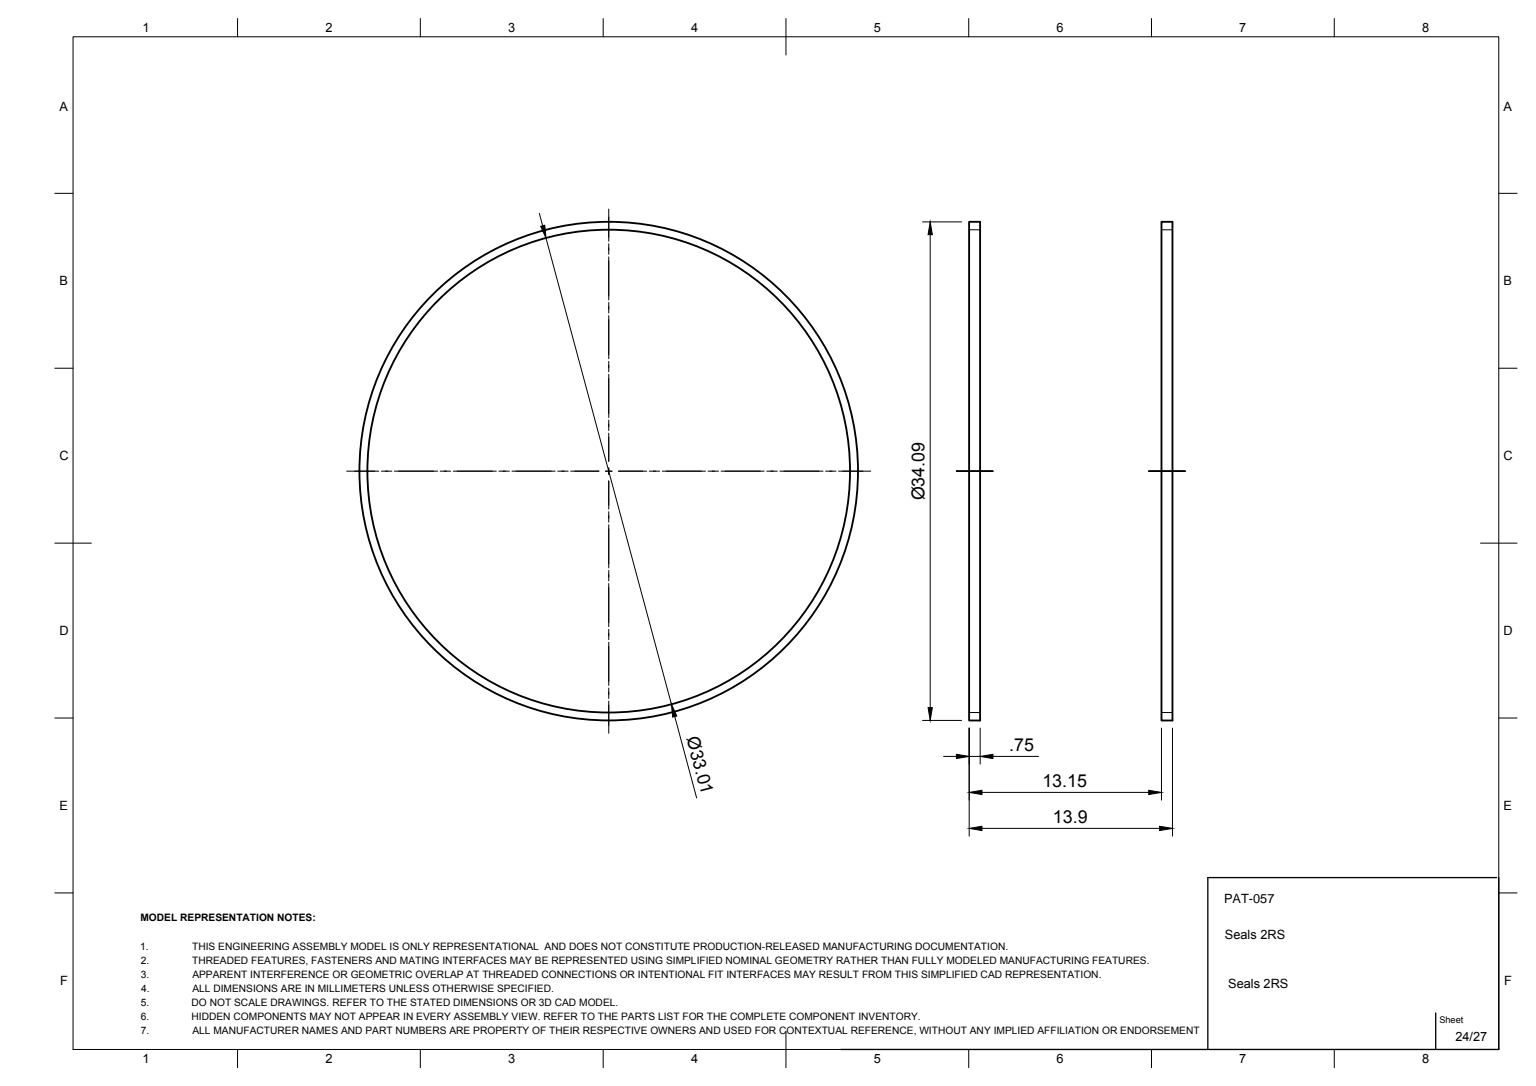
ISO-10303-21;
HEADER;
/* Generated by software containing ST-Developer
 * from STEP Tools, Inc. (www.steptools.com) 
 */

FILE_DESCRIPTION(
/* description */ ('Bearing-mounted hook block'),
/* implementation_level */ '2;1');

FILE_NAME(
/* name */ 'Seals 2RS.step',
/* time_stamp */ '2026-10-28T22:30:11-07:00',
/* author */ (''),
/* organization */ (''),
/* preprocessor_version */ 'ST-DEVELOPER v20.2',
/* originating_system */ 'Autodesk Translation Framework v15.17.0.0',
/* authorisation */ '');

FILE_SCHEMA (('AUTOMOTIVE_DESIGN { 1 0 10303 214 3 1 1 }'));
ENDSEC;

DATA;
#10=MECHANICAL_DESIGN_GEOMETRIC_PRESENTATION_REPRESENTATION('',(#348,#349),#7609);
#293=SHAPE_REPRESENTATION_RELATIONSHIP('SRR','None',#7742,#317);
#317=ADVANCED_BREP_SHAPE_REPRESENTATION('',(#378,#379),#7602);
#348=STYLED_ITEM('',(#7931),#378);
#349=STYLED_ITEM('',(#7931),#379);
#378=MANIFOLD_SOLID_BREP('Body1',#3946);
#379=MANIFOLD_SOLID_BREP('Body2',#3947);
#537=LINE('',#7259,#767);
#538=LINE('',#7264,#768);
#539=LINE('',#7273,#769);
#540=LINE('',#7278,#770);
#767=VECTOR('',#5714,1.70469);
#768=VECTOR('',#5721,1.65031);
#769=VECTOR('',#5732,1.70469);
#770=VECTOR('',#5739,1.65031);
#900=CYLINDRICAL_SURFACE('',#4619,1.70469);
#901=CYLINDRICAL_SURFACE('',#4623,1.65031);
#902=CYLINDRICAL_SURFACE('',#4627,1.70469);
#903=CYLINDRICAL_SURFACE('',#4631,1.65031);
#979=FACE_BOUND('',#1469,.T.);
#980=FACE_BOUND('',#1472,.T.);
#981=FACE_BOUND('',#1475,.T.);
#982=FACE_BOUND('',#1478,.T.);
#1174=FACE_OUTER_BOUND('',#1468,.T.);
#1175=FACE_OUTER_BOUND('',#1470,.T.);
#1176=FACE_OUTER_BOUND('',#1471,.T.);
#1177=FACE_OUTER_BOUND('',#1473,.T.);
#1178=FACE_OUTER_BOUND('',#1474,.T.);
#1179=FACE_OUTER_BOUND('',#1476,.T.);
#1180=FACE_OUTER_BOUND('',#1477,.T.);
#1181=FACE_OUTER_BOUND('',#1479,.T.);
#1468=EDGE_LOOP('',(#3312));
#1469=EDGE_LOOP('',(#3313));
#1470=EDGE_LOOP('',(#3314,#3315,#3316,#3317));
#1471=EDGE_LOOP('',(#3318));
#1472=EDGE_LOOP('',(#3319));
#1473=EDGE_LOOP('',(#3320,#3321,#3322,#3323));
#1474=EDGE_LOOP('',(#3324));
#1475=EDGE_LOOP('',(#3325));
#1476=EDGE_LOOP('',(#3326,#3327,#3328,#3329));
#1477=EDGE_LOOP('',(#3330));
#1478=EDGE_LOOP('',(#3331));
#1479=EDGE_LOOP('',(#3332,#3333,#3334,#3335));
#1731=CIRCLE('',#4617,1.70469);
#1732=CIRCLE('',#4618,1.65031);
#1733=CIRCLE('',#4620,1.70469);
#1734=CIRCLE('',#4622,1.65031);
#1735=CIRCLE('',#4625,1.70469);
#1736=CIRCLE('',#4626,1.65031);
#1737=CIRCLE('',#4628,1.70469);
#1738=CIRCLE('',#4630,1.65031);
#2024=VERTEX_POINT('',#7252);
#2025=VERTEX_POINT('',#7254);
#2026=VERTEX_POINT('',#7257);
#2027=VERTEX_POINT('',#7261);
#2028=VERTEX_POINT('',#7266);
#2029=VERTEX_POINT('',#7268);
#2030=VERTEX_POINT('',#7271);
#2031=VERTEX_POINT('',#7275);
#2466=EDGE_CURVE('',#2024,#2024,#1731,.T.);
#2467=EDGE_CURVE('',#2025,#2025,#1732,.T.);
#2468=EDGE_CURVE('',#2026,#2026,#1733,.T.);
#2469=EDGE_CURVE('',#2026,#2024,#537,.T.);
#2470=EDGE_CURVE('',#2027,#2027,#1734,.T.);
#2471=EDGE_CURVE('',#2027,#2025,#538,.T.);
#2472=EDGE_CURVE('',#2028,#2028,#1735,.T.);
#2473=EDGE_CURVE('',#2029,#2029,#1736,.T.);
#2474=EDGE_CURVE('',#2030,#2030,#1737,.T.);
#2475=EDGE_CURVE('',#2030,#2028,#539,.T.);
#2476=EDGE_CURVE('',#2031,#2031,#1738,.T.);
#2477=EDGE_CURVE('',#2031,#2029,#540,.T.);
#3312=ORIENTED_EDGE('',*,*,#2466,.F.);
#3313=ORIENTED_EDGE('',*,*,#2467,.T.);
#3314=ORIENTED_EDGE('',*,*,#2468,.F.);
#3315=ORIENTED_EDGE('',*,*,#2469,.T.);
#3316=ORIENTED_EDGE('',*,*,#2466,.T.);
#3317=ORIENTED_EDGE('',*,*,#2469,.F.);
#3318=ORIENTED_EDGE('',*,*,#2468,.T.);
#3319=ORIENTED_EDGE('',*,*,#2470,.F.);
#3320=ORIENTED_EDGE('',*,*,#2470,.T.);
#3321=ORIENTED_EDGE('',*,*,#2471,.T.);
#3322=ORIENTED_EDGE('',*,*,#2467,.F.);
#3323=ORIENTED_EDGE('',*,*,#2471,.F.);
#3324=ORIENTED_EDGE('',*,*,#2472,.F.);
#3325=ORIENTED_EDGE('',*,*,#2473,.T.);
#3326=ORIENTED_EDGE('',*,*,#2474,.F.);
#3327=ORIENTED_EDGE('',*,*,#2475,.T.);
#3328=ORIENTED_EDGE('',*,*,#2472,.T.);
#3329=ORIENTED_EDGE('',*,*,#2475,.F.);
#3330=ORIENTED_EDGE('',*,*,#2474,.T.);
#3331=ORIENTED_EDGE('',*,*,#2476,.F.);
#3332=ORIENTED_EDGE('',*,*,#2476,.T.);
#3333=ORIENTED_EDGE('',*,*,#2477,.T.);
#3334=ORIENTED_EDGE('',*,*,#2473,.F.);
#3335=ORIENTED_EDGE('',*,*,#2477,.F.);
#3644=PLANE('',#4616);
#3645=PLANE('',#4621);
#3646=PLANE('',#4624);
#3647=PLANE('',#4629);
#3856=ADVANCED_FACE('',(#1174,#979),#3644,.T.);
#3857=ADVANCED_FACE('',(#1175),#900,.T.);
#3858=ADVANCED_FACE('',(#1176,#980),#3645,.T.);
#3859=ADVANCED_FACE('',(#1177),#901,.F.);
#3860=ADVANCED_FACE('',(#1178,#981),#3646,.T.);
#3861=ADVANCED_FACE('',(#1179),#902,.T.);
#3862=ADVANCED_FACE('',(#1180,#982),#3647,.T.);
#3863=ADVANCED_FACE('',(#1181),#903,.F.);
#3946=CLOSED_SHELL('',(#3856,#3857,#3858,#3859));
#3947=CLOSED_SHELL('',(#3860,#3861,#3862,#3863));
#4615=AXIS2_PLACEMENT_3D('',#7250,#5702,#5703);
#4616=AXIS2_PLACEMENT_3D('',#7251,#5704,#5705);
#4617=AXIS2_PLACEMENT_3D('',#7253,#5706,#5707);
#4618=AXIS2_PLACEMENT_3D('',#7255,#5708,#5709);
#4619=AXIS2_PLACEMENT_3D('',#7256,#5710,#5711);
#4620=AXIS2_PLACEMENT_3D('',#7258,#5712,#5713);
#4621=AXIS2_PLACEMENT_3D('',#7260,#5715,#5716);
#4622=AXIS2_PLACEMENT_3D('',#7262,#5717,#5718);
#4623=AXIS2_PLACEMENT_3D('',#7263,#5719,#5720);
#4624=AXIS2_PLACEMENT_3D('',#7265,#5722,#5723);
#4625=AXIS2_PLACEMENT_3D('',#7267,#5724,#5725);
#4626=AXIS2_PLACEMENT_3D('',#7269,#5726,#5727);
#4627=AXIS2_PLACEMENT_3D('',#7270,#5728,#5729);
#4628=AXIS2_PLACEMENT_3D('',#7272,#5730,#5731);
#4629=AXIS2_PLACEMENT_3D('',#7274,#5733,#5734);
#4630=AXIS2_PLACEMENT_3D('',#7276,#5735,#5736);
#4631=AXIS2_PLACEMENT_3D('',#7277,#5737,#5738);
#5702=DIRECTION('axis',(0.,0.,1.));
#5703=DIRECTION('refdir',(1.,0.,0.));
#5704=DIRECTION('center_axis',(0.,1.,0.));
#5705=DIRECTION('ref_axis',(0.,0.,1.));
#5706=DIRECTION('center_axis',(0.,-1.,0.));
#5707=DIRECTION('ref_axis',(1.,0.,0.));
#5708=DIRECTION('center_axis',(0.,-1.,0.));
#5709=DIRECTION('ref_axis',(1.,0.,0.));
#5710=DIRECTION('center_axis',(0.,-1.,0.));
#5711=DIRECTION('ref_axis',(1.,0.,0.));
#5712=DIRECTION('center_axis',(0.,-1.,0.));
#5713=DIRECTION('ref_axis',(1.,0.,0.));
#5714=DIRECTION('',(0.,1.,0.));
#5715=DIRECTION('center_axis',(0.,-1.,0.));
#5716=DIRECTION('ref_axis',(0.,0.,-1.));
#5717=DIRECTION('center_axis',(0.,-1.,0.));
#5718=DIRECTION('ref_axis',(1.,0.,0.));
#5719=DIRECTION('center_axis',(0.,-1.,0.));
#5720=DIRECTION('ref_axis',(1.,0.,0.));
#5721=DIRECTION('',(0.,1.,0.));
#5722=DIRECTION('center_axis',(0.,1.,0.));
#5723=DIRECTION('ref_axis',(0.,0.,1.));
#5724=DIRECTION('center_axis',(0.,-1.,0.));
#5725=DIRECTION('ref_axis',(1.,0.,0.));
#5726=DIRECTION('center_axis',(0.,-1.,0.));
#5727=DIRECTION('ref_axis',(1.,0.,0.));
#5728=DIRECTION('center_axis',(0.,-1.,0.));
#5729=DIRECTION('ref_axis',(1.,0.,0.));
#5730=DIRECTION('center_axis',(0.,-1.,0.));
#5731=DIRECTION('ref_axis',(1.,0.,0.));
#5732=DIRECTION('',(0.,1.,0.));
#5733=DIRECTION('center_axis',(0.,-1.,0.));
#5734=DIRECTION('ref_axis',(0.,0.,-1.));
#5735=DIRECTION('center_axis',(0.,-1.,0.));
#5736=DIRECTION('ref_axis',(1.,0.,0.));
#5737=DIRECTION('center_axis',(0.,-1.,0.));
#5738=DIRECTION('ref_axis',(1.,0.,0.));
#5739=DIRECTION('',(0.,1.,0.));
#7250=CARTESIAN_POINT('',(0.,0.,0.));
#7251=CARTESIAN_POINT('Origin',(1.70469,0.695,0.));
#7252=CARTESIAN_POINT('',(-1.70469,0.695,-2.0876431520385E-16));
#7253=CARTESIAN_POINT('Origin',(0.,0.695,0.));
#7254=CARTESIAN_POINT('',(-1.65031,0.695,-2.02104685910087E-16));
#7255=CARTESIAN_POINT('Origin',(0.,0.695,0.));
#7256=CARTESIAN_POINT('Origin',(0.,0.6575,0.));
#7257=CARTESIAN_POINT('',(-1.70469,0.62,-2.0876431520385E-16));
#7258=CARTESIAN_POINT('Origin',(0.,0.62,0.));
#7259=CARTESIAN_POINT('',(-1.70469,0.6575,-2.0876431520385E-16));
#7260=CARTESIAN_POINT('Origin',(1.65031,0.62,0.));
#7261=CARTESIAN_POINT('',(-1.65031,0.62,-2.02104685910087E-16));
#7262=CARTESIAN_POINT('Origin',(0.,0.62,0.));
#7263=CARTESIAN_POINT('Origin',(0.,0.6575,0.));
#7264=CARTESIAN_POINT('',(-1.65031,0.6575,-2.02104685910087E-16));
#7265=CARTESIAN_POINT('Origin',(1.70469,-0.62,0.));
#7266=CARTESIAN_POINT('',(-1.70469,-0.62,-2.0876431520385E-16));
#7267=CARTESIAN_POINT('Origin',(0.,-0.62,0.));
#7268=CARTESIAN_POINT('',(-1.65031,-0.62,-2.02104685910087E-16));
#7269=CARTESIAN_POINT('Origin',(0.,-0.62,0.));
#7270=CARTESIAN_POINT('Origin',(0.,-0.6575,0.));
#7271=CARTESIAN_POINT('',(-1.70469,-0.695,-2.0876431520385E-16));
#7272=CARTESIAN_POINT('Origin',(0.,-0.695,0.));
#7273=CARTESIAN_POINT('',(-1.70469,-0.6575,-2.0876431520385E-16));
#7274=CARTESIAN_POINT('Origin',(1.65031,-0.695,0.));
#7275=CARTESIAN_POINT('',(-1.65031,-0.695,-2.02104685910087E-16));
#7276=CARTESIAN_POINT('Origin',(0.,-0.695,0.));
#7277=CARTESIAN_POINT('Origin',(0.,-0.6575,0.));
#7278=CARTESIAN_POINT('',(-1.65031,-0.6575,-2.02104685910087E-16));
#7572=UNCERTAINTY_MEASURE_WITH_UNIT(LENGTH_MEASURE(0.001),#7610,
'DISTANCE_ACCURACY_VALUE',
'Maximum model space distance between geometric entities at asserted c
onnectivities');
#7579=UNCERTAINTY_MEASURE_WITH_UNIT(LENGTH_MEASURE(0.001),#7610,
'DISTANCE_ACCURACY_VALUE',
'Maximum model space distance between geometric entities at asserted c
onnectivities');
#7602=(
GEOMETRIC_REPRESENTATION_CONTEXT(3)
GLOBAL_UNCERTAINTY_ASSIGNED_CONTEXT((#7572))
GLOBAL_UNIT_ASSIGNED_CONTEXT((#7610,#7612,#7613))
REPRESENTATION_CONTEXT('','3D')
);
#7609=(
GEOMETRIC_REPRESENTATION_CONTEXT(3)
GLOBAL_UNCERTAINTY_ASSIGNED_CONTEXT((#7579))
GLOBAL_UNIT_ASSIGNED_CONTEXT((#7610,#7612,#7613))
REPRESENTATION_CONTEXT('','3D')
);
#7610=(
LENGTH_UNIT()
NAMED_UNIT(*)
SI_UNIT(.CENTI.,.METRE.)
);
#7612=(
NAMED_UNIT(*)
PLANE_ANGLE_UNIT()
SI_UNIT($,.RADIAN.)
);
#7613=(
NAMED_UNIT(*)
SI_UNIT($,.STERADIAN.)
SOLID_ANGLE_UNIT()
);
#7636=SHAPE_DEFINITION_REPRESENTATION(#7688,#7742);
#7688=PRODUCT_DEFINITION_SHAPE('',$,#7772);
#7742=SHAPE_REPRESENTATION('',(#4615),#7602);
#7749=PRODUCT_DEFINITION_CONTEXT('part definition',#7838,'design');
#7772=PRODUCT_DEFINITION('Seals 2RS','Seals 2RS',#7801,#7749);
#7801=PRODUCT_DEFINITION_FORMATION('',$,#7862);
#7838=APPLICATION_CONTEXT(
'Core Data for Automotive Mechanical Design Process');
#7839=PRODUCT_CONTEXT('part definition',#7838,'mechanical');
#7862=PRODUCT('Seals 2RS','Seals 2RS','Seals 2RS',(#7839));
#7925=COLOUR_RGB('Grey',0.48,0.52,0.57);
#7926=FILL_AREA_STYLE_COLOUR('',#7925);
#7927=FILL_AREA_STYLE('',(#7926));
#7928=SURFACE_STYLE_FILL_AREA(#7927);
#7929=SURFACE_SIDE_STYLE('',(#7928));
#7930=SURFACE_STYLE_USAGE(.BOTH.,#7929);
#7931=PRESENTATION_STYLE_ASSIGNMENT((#7930));
ENDSEC;
END-ISO-10303-21;
